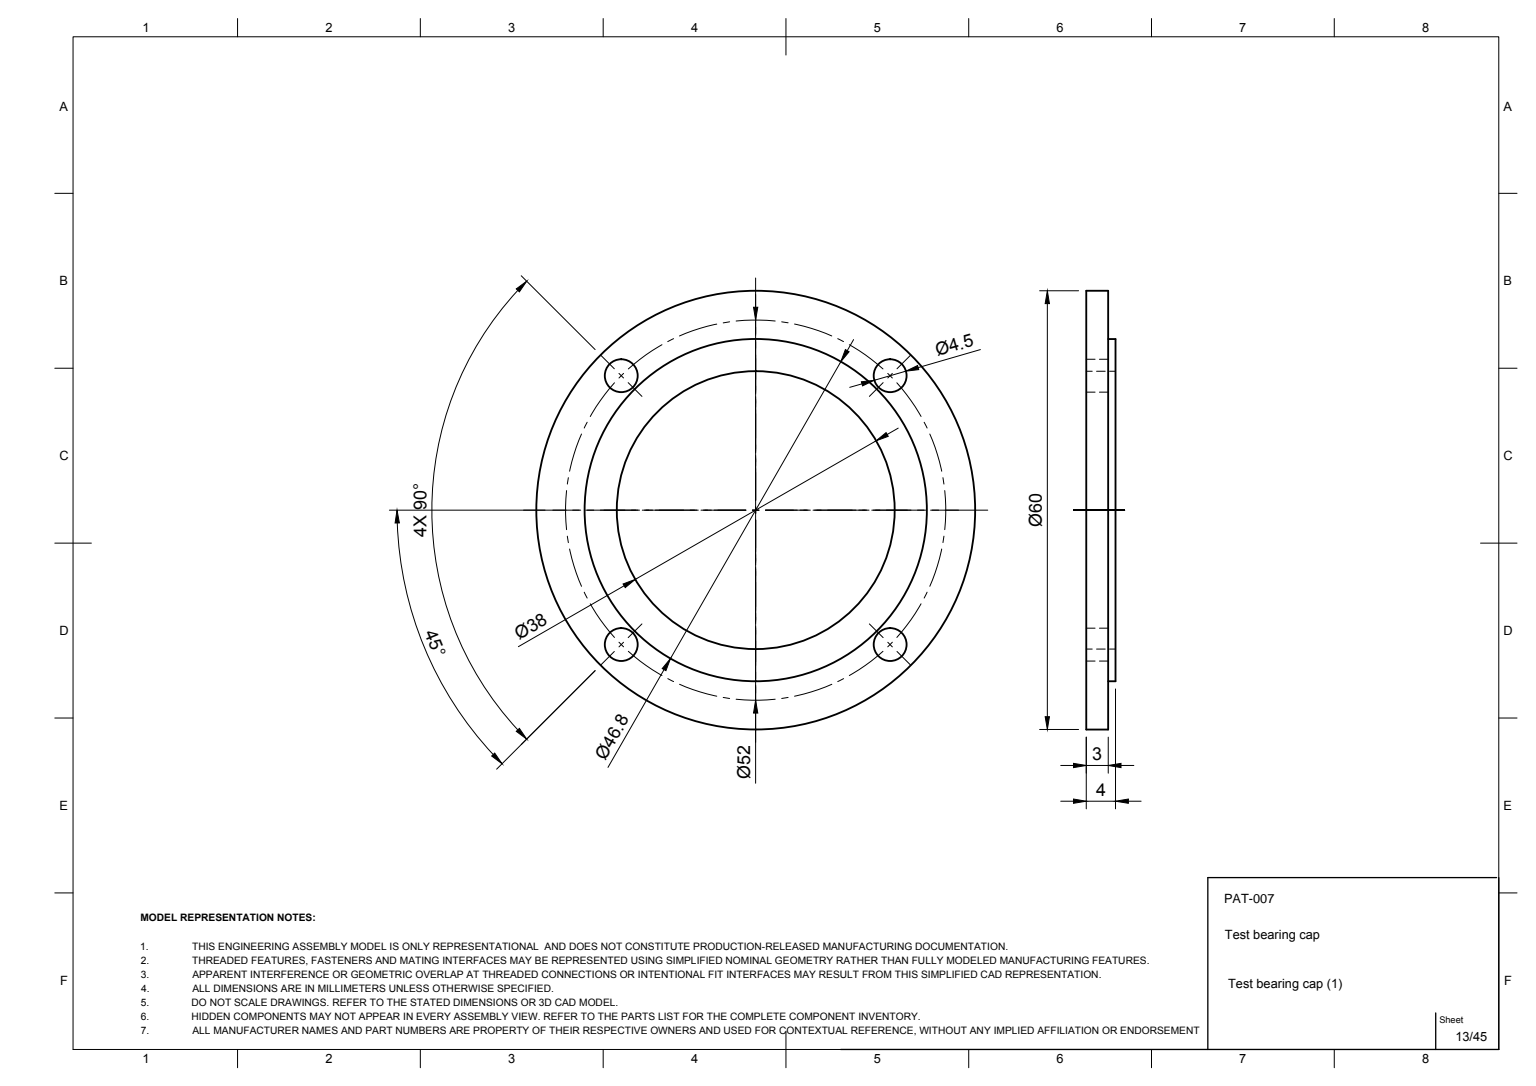
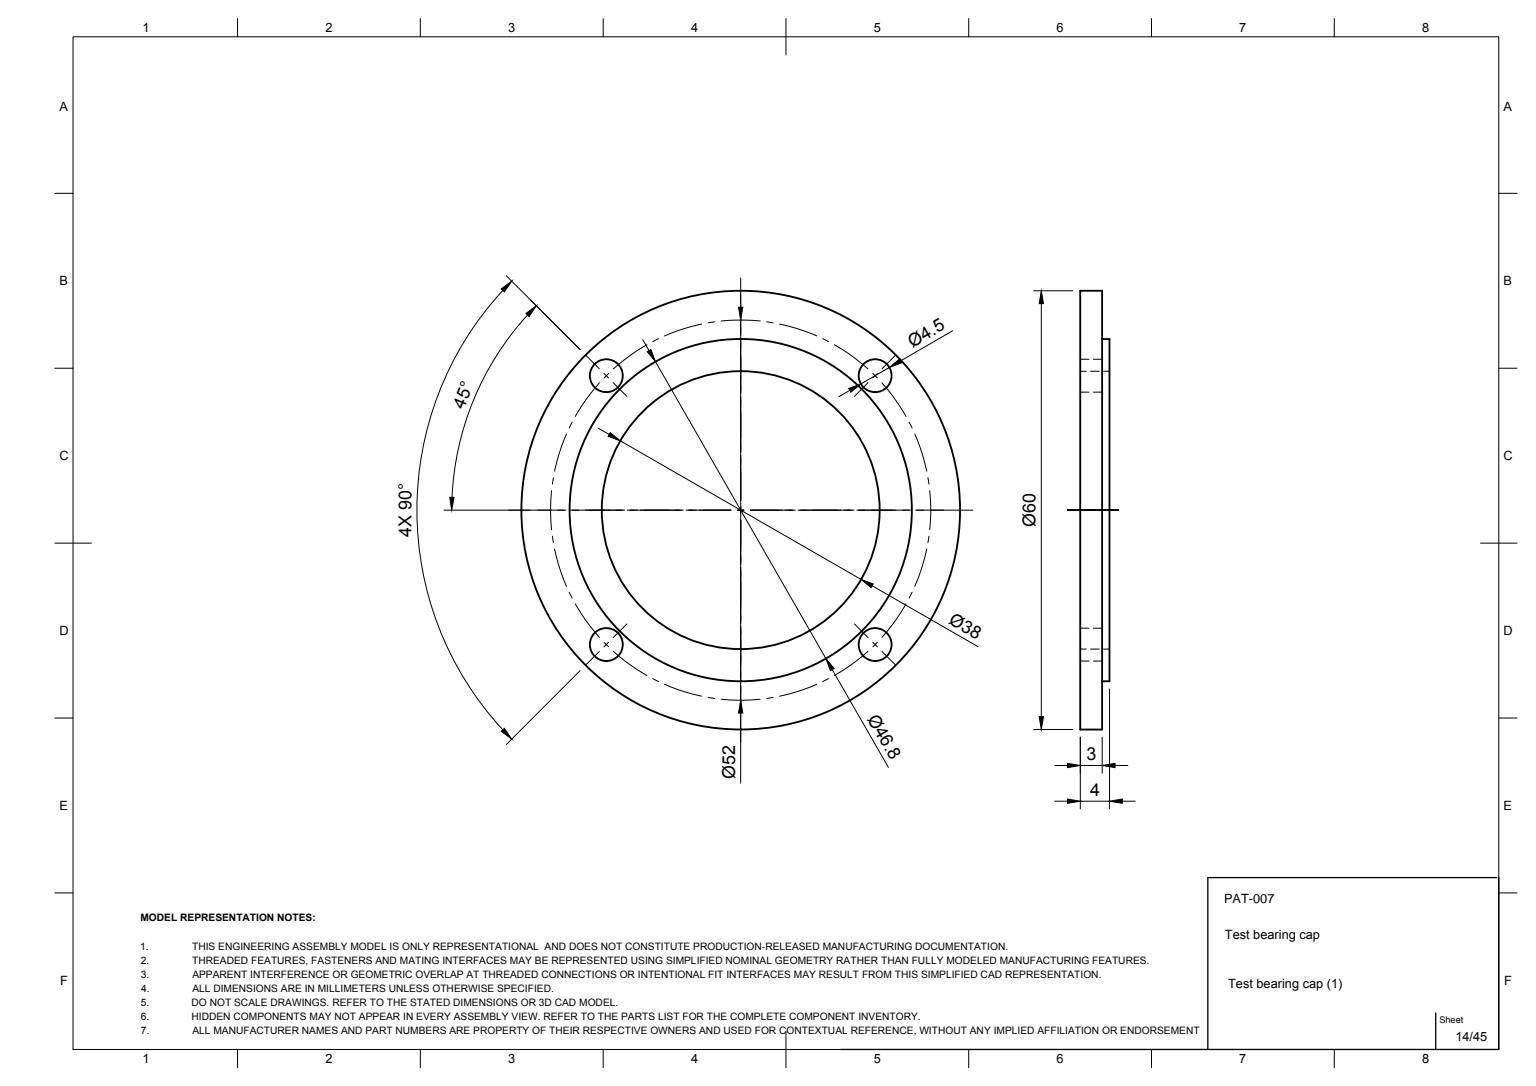
ISO-10303-21;
HEADER;
/* Generated by software containing ST-Developer
 * from STEP Tools, Inc. (www.steptools.com) 
 */

FILE_DESCRIPTION(
/* description */ ('Bearing friction torque test rig'),
/* implementation_level */ '2;1');

FILE_NAME(
/* name */ 'Test bearing cap.step',
/* time_stamp */ '2026-10-28T03:24:04-07:00',
/* author */ (''),
/* organization */ (''),
/* preprocessor_version */ 'ST-DEVELOPER v20.2',
/* originating_system */ 'Autodesk Translation Framework v15.17.0.0',
/* authorisation */ '');

FILE_SCHEMA (('AUTOMOTIVE_DESIGN { 1 0 10303 214 3 1 1 }'));
ENDSEC;

DATA;
#10=MECHANICAL_DESIGN_GEOMETRIC_PRESENTATION_REPRESENTATION('',(#547),#14822);
#469=SHAPE_REPRESENTATION_RELATIONSHIP('SRR','None',#15008,#508);
#508=ADVANCED_BREP_SHAPE_REPRESENTATION('',(#601),#14788);
#547=STYLED_ITEM('',(#15284),#601);
#601=MANIFOLD_SOLID_BREP('Body1',#7663);
#755=FACE_BOUND('',#1774,.T.);
#756=FACE_BOUND('',#1778,.T.);
#757=FACE_BOUND('',#1779,.T.);
#758=FACE_BOUND('',#1780,.T.);
#759=FACE_BOUND('',#1781,.T.);
#760=FACE_BOUND('',#1782,.T.);
#761=FACE_BOUND('',#1784,.T.);
#762=FACE_BOUND('',#1785,.T.);
#763=FACE_BOUND('',#1786,.T.);
#764=FACE_BOUND('',#1787,.T.);
#765=FACE_BOUND('',#1788,.T.);
#921=PLANE('',#8423);
#922=PLANE('',#8430);
#923=PLANE('',#8431);
#1212=FACE_OUTER_BOUND('',#1768,.T.);
#1213=FACE_OUTER_BOUND('',#1769,.T.);
#1214=FACE_OUTER_BOUND('',#1770,.T.);
#1215=FACE_OUTER_BOUND('',#1771,.T.);
#1216=FACE_OUTER_BOUND('',#1772,.T.);
#1217=FACE_OUTER_BOUND('',#1773,.T.);
#1218=FACE_OUTER_BOUND('',#1775,.T.);
#1219=FACE_OUTER_BOUND('',#1776,.T.);
#1220=FACE_OUTER_BOUND('',#1777,.T.);
#1221=FACE_OUTER_BOUND('',#1783,.T.);
#1768=EDGE_LOOP('',(#5676,#5677,#5678,#5679));
#1769=EDGE_LOOP('',(#5680,#5681,#5682,#5683));
#1770=EDGE_LOOP('',(#5684,#5685,#5686,#5687));
#1771=EDGE_LOOP('',(#5688,#5689,#5690,#5691));
#1772=EDGE_LOOP('',(#5692,#5693,#5694,#5695));
#1773=EDGE_LOOP('',(#5696));
#1774=EDGE_LOOP('',(#5697));
#1775=EDGE_LOOP('',(#5698,#5699,#5700,#5701));
#1776=EDGE_LOOP('',(#5702,#5703,#5704,#5705));
#1777=EDGE_LOOP('',(#5706));
#1778=EDGE_LOOP('',(#5707));
#1779=EDGE_LOOP('',(#5708));
#1780=EDGE_LOOP('',(#5709));
#1781=EDGE_LOOP('',(#5710));
#1782=EDGE_LOOP('',(#5711));
#1783=EDGE_LOOP('',(#5712));
#1784=EDGE_LOOP('',(#5713));
#1785=EDGE_LOOP('',(#5714));
#1786=EDGE_LOOP('',(#5715));
#1787=EDGE_LOOP('',(#5716));
#1788=EDGE_LOOP('',(#5717));
#2341=LINE('',#12226,#2785);
#2342=LINE('',#12232,#2786);
#2343=LINE('',#12238,#2787);
#2344=LINE('',#12244,#2788);
#2345=LINE('',#12250,#2789);
#2346=LINE('',#12257,#2790);
#2347=LINE('',#12263,#2791);
#2785=VECTOR('',#9824,0.225);
#2786=VECTOR('',#9831,0.225);
#2787=VECTOR('',#9838,0.225);
#2788=VECTOR('',#9845,0.225);
#2789=VECTOR('',#9852,2.34);
#2790=VECTOR('',#9861,1.9);
#2791=VECTOR('',#9868,3.);
#3243=CIRCLE('',#8409,0.225);
#3244=CIRCLE('',#8410,0.225);
#3245=CIRCLE('',#8412,0.225);
#3246=CIRCLE('',#8413,0.225);
#3247=CIRCLE('',#8415,0.225);
#3248=CIRCLE('',#8416,0.225);
#3249=CIRCLE('',#8418,0.225);
#3250=CIRCLE('',#8419,0.225);
#3251=CIRCLE('',#8421,2.34);
#3252=CIRCLE('',#8422,2.34);
#3253=CIRCLE('',#8424,1.9);
#3254=CIRCLE('',#8426,1.9);
#3255=CIRCLE('',#8428,3.);
#3256=CIRCLE('',#8429,3.);
#3729=VERTEX_POINT('',#12223);
#3730=VERTEX_POINT('',#12225);
#3731=VERTEX_POINT('',#12229);
#3732=VERTEX_POINT('',#12231);
#3733=VERTEX_POINT('',#12235);
#3734=VERTEX_POINT('',#12237);
#3735=VERTEX_POINT('',#12241);
#3736=VERTEX_POINT('',#12243);
#3737=VERTEX_POINT('',#12247);
#3738=VERTEX_POINT('',#12249);
#3739=VERTEX_POINT('',#12253);
#3740=VERTEX_POINT('',#12256);
#3741=VERTEX_POINT('',#12260);
#3742=VERTEX_POINT('',#12262);
#4464=EDGE_CURVE('',#3729,#3729,#3243,.T.);
#4465=EDGE_CURVE('',#3729,#3730,#2341,.T.);
#4466=EDGE_CURVE('',#3730,#3730,#3244,.T.);
#4467=EDGE_CURVE('',#3731,#3731,#3245,.T.);
#4468=EDGE_CURVE('',#3731,#3732,#2342,.T.);
#4469=EDGE_CURVE('',#3732,#3732,#3246,.T.);
#4470=EDGE_CURVE('',#3733,#3733,#3247,.T.);
#4471=EDGE_CURVE('',#3733,#3734,#2343,.T.);
#4472=EDGE_CURVE('',#3734,#3734,#3248,.T.);
#4473=EDGE_CURVE('',#3735,#3735,#3249,.T.);
#4474=EDGE_CURVE('',#3735,#3736,#2344,.T.);
#4475=EDGE_CURVE('',#3736,#3736,#3250,.T.);
#4476=EDGE_CURVE('',#3737,#3737,#3251,.T.);
#4477=EDGE_CURVE('',#3737,#3738,#2345,.T.);
#4478=EDGE_CURVE('',#3738,#3738,#3252,.T.);
#4479=EDGE_CURVE('',#3739,#3739,#3253,.T.);
#4480=EDGE_CURVE('',#3739,#3740,#2346,.T.);
#4481=EDGE_CURVE('',#3740,#3740,#3254,.T.);
#4482=EDGE_CURVE('',#3741,#3741,#3255,.T.);
#4483=EDGE_CURVE('',#3741,#3742,#2347,.T.);
#4484=EDGE_CURVE('',#3742,#3742,#3256,.T.);
#5676=ORIENTED_EDGE('',*,*,#4464,.F.);
#5677=ORIENTED_EDGE('',*,*,#4465,.T.);
#5678=ORIENTED_EDGE('',*,*,#4466,.F.);
#5679=ORIENTED_EDGE('',*,*,#4465,.F.);
#5680=ORIENTED_EDGE('',*,*,#4467,.F.);
#5681=ORIENTED_EDGE('',*,*,#4468,.T.);
#5682=ORIENTED_EDGE('',*,*,#4469,.F.);
#5683=ORIENTED_EDGE('',*,*,#4468,.F.);
#5684=ORIENTED_EDGE('',*,*,#4470,.F.);
#5685=ORIENTED_EDGE('',*,*,#4471,.T.);
#5686=ORIENTED_EDGE('',*,*,#4472,.F.);
#5687=ORIENTED_EDGE('',*,*,#4471,.F.);
#5688=ORIENTED_EDGE('',*,*,#4473,.F.);
#5689=ORIENTED_EDGE('',*,*,#4474,.T.);
#5690=ORIENTED_EDGE('',*,*,#4475,.F.);
#5691=ORIENTED_EDGE('',*,*,#4474,.F.);
#5692=ORIENTED_EDGE('',*,*,#4476,.F.);
#5693=ORIENTED_EDGE('',*,*,#4477,.T.);
#5694=ORIENTED_EDGE('',*,*,#4478,.F.);
#5695=ORIENTED_EDGE('',*,*,#4477,.F.);
#5696=ORIENTED_EDGE('',*,*,#4476,.T.);
#5697=ORIENTED_EDGE('',*,*,#4479,.T.);
#5698=ORIENTED_EDGE('',*,*,#4479,.F.);
#5699=ORIENTED_EDGE('',*,*,#4480,.T.);
#5700=ORIENTED_EDGE('',*,*,#4481,.T.);
#5701=ORIENTED_EDGE('',*,*,#4480,.F.);
#5702=ORIENTED_EDGE('',*,*,#4482,.F.);
#5703=ORIENTED_EDGE('',*,*,#4483,.T.);
#5704=ORIENTED_EDGE('',*,*,#4484,.T.);
#5705=ORIENTED_EDGE('',*,*,#4483,.F.);
#5706=ORIENTED_EDGE('',*,*,#4482,.T.);
#5707=ORIENTED_EDGE('',*,*,#4478,.T.);
#5708=ORIENTED_EDGE('',*,*,#4475,.T.);
#5709=ORIENTED_EDGE('',*,*,#4472,.T.);
#5710=ORIENTED_EDGE('',*,*,#4469,.T.);
#5711=ORIENTED_EDGE('',*,*,#4466,.T.);
#5712=ORIENTED_EDGE('',*,*,#4484,.F.);
#5713=ORIENTED_EDGE('',*,*,#4481,.F.);
#5714=ORIENTED_EDGE('',*,*,#4473,.T.);
#5715=ORIENTED_EDGE('',*,*,#4470,.T.);
#5716=ORIENTED_EDGE('',*,*,#4467,.T.);
#5717=ORIENTED_EDGE('',*,*,#4464,.T.);
#7110=CYLINDRICAL_SURFACE('',#8408,0.225);
#7111=CYLINDRICAL_SURFACE('',#8411,0.225);
#7112=CYLINDRICAL_SURFACE('',#8414,0.225);
#7113=CYLINDRICAL_SURFACE('',#8417,0.225);
#7114=CYLINDRICAL_SURFACE('',#8420,2.34);
#7115=CYLINDRICAL_SURFACE('',#8425,1.9);
#7116=CYLINDRICAL_SURFACE('',#8427,3.);
#7323=ADVANCED_FACE('',(#1212),#7110,.F.);
#7324=ADVANCED_FACE('',(#1213),#7111,.F.);
#7325=ADVANCED_FACE('',(#1214),#7112,.F.);
#7326=ADVANCED_FACE('',(#1215),#7113,.F.);
#7327=ADVANCED_FACE('',(#1216),#7114,.T.);
#7328=ADVANCED_FACE('',(#1217,#755),#921,.T.);
#7329=ADVANCED_FACE('',(#1218),#7115,.F.);
#7330=ADVANCED_FACE('',(#1219),#7116,.T.);
#7331=ADVANCED_FACE('',(#1220,#756,#757,#758,#759,#760),#922,.T.);
#7332=ADVANCED_FACE('',(#1221,#761,#762,#763,#764,#765),#923,.F.);
#7663=CLOSED_SHELL('',(#7323,#7324,#7325,#7326,#7327,#7328,#7329,#7330,
#7331,#7332));
#8407=AXIS2_PLACEMENT_3D('',#12221,#9818,#9819);
#8408=AXIS2_PLACEMENT_3D('',#12222,#9820,#9821);
#8409=AXIS2_PLACEMENT_3D('',#12224,#9822,#9823);
#8410=AXIS2_PLACEMENT_3D('',#12227,#9825,#9826);
#8411=AXIS2_PLACEMENT_3D('',#12228,#9827,#9828);
#8412=AXIS2_PLACEMENT_3D('',#12230,#9829,#9830);
#8413=AXIS2_PLACEMENT_3D('',#12233,#9832,#9833);
#8414=AXIS2_PLACEMENT_3D('',#12234,#9834,#9835);
#8415=AXIS2_PLACEMENT_3D('',#12236,#9836,#9837);
#8416=AXIS2_PLACEMENT_3D('',#12239,#9839,#9840);
#8417=AXIS2_PLACEMENT_3D('',#12240,#9841,#9842);
#8418=AXIS2_PLACEMENT_3D('',#12242,#9843,#9844);
#8419=AXIS2_PLACEMENT_3D('',#12245,#9846,#9847);
#8420=AXIS2_PLACEMENT_3D('',#12246,#9848,#9849);
#8421=AXIS2_PLACEMENT_3D('',#12248,#9850,#9851);
#8422=AXIS2_PLACEMENT_3D('',#12251,#9853,#9854);
#8423=AXIS2_PLACEMENT_3D('',#12252,#9855,#9856);
#8424=AXIS2_PLACEMENT_3D('',#12254,#9857,#9858);
#8425=AXIS2_PLACEMENT_3D('',#12255,#9859,#9860);
#8426=AXIS2_PLACEMENT_3D('',#12258,#9862,#9863);
#8427=AXIS2_PLACEMENT_3D('',#12259,#9864,#9865);
#8428=AXIS2_PLACEMENT_3D('',#12261,#9866,#9867);
#8429=AXIS2_PLACEMENT_3D('',#12264,#9869,#9870);
#8430=AXIS2_PLACEMENT_3D('',#12265,#9871,#9872);
#8431=AXIS2_PLACEMENT_3D('',#12266,#9873,#9874);
#9818=DIRECTION('axis',(0.,0.,1.));
#9819=DIRECTION('refdir',(1.,0.,0.));
#9820=DIRECTION('center_axis',(0.,1.,0.));
#9821=DIRECTION('ref_axis',(1.,0.,0.));
#9822=DIRECTION('center_axis',(0.,1.,0.));
#9823=DIRECTION('ref_axis',(1.,0.,0.));
#9824=DIRECTION('',(0.,1.,0.));
#9825=DIRECTION('center_axis',(0.,-1.,0.));
#9826=DIRECTION('ref_axis',(1.,0.,0.));
#9827=DIRECTION('center_axis',(0.,1.,0.));
#9828=DIRECTION('ref_axis',(1.,0.,0.));
#9829=DIRECTION('center_axis',(0.,1.,0.));
#9830=DIRECTION('ref_axis',(1.,0.,0.));
#9831=DIRECTION('',(0.,1.,0.));
#9832=DIRECTION('center_axis',(0.,-1.,0.));
#9833=DIRECTION('ref_axis',(1.,0.,0.));
#9834=DIRECTION('center_axis',(0.,1.,0.));
#9835=DIRECTION('ref_axis',(1.,0.,0.));
#9836=DIRECTION('center_axis',(0.,1.,0.));
#9837=DIRECTION('ref_axis',(1.,0.,0.));
#9838=DIRECTION('',(0.,1.,0.));
#9839=DIRECTION('center_axis',(0.,-1.,0.));
#9840=DIRECTION('ref_axis',(1.,0.,0.));
#9841=DIRECTION('center_axis',(0.,1.,0.));
#9842=DIRECTION('ref_axis',(1.,0.,0.));
#9843=DIRECTION('center_axis',(0.,1.,0.));
#9844=DIRECTION('ref_axis',(1.,0.,0.));
#9845=DIRECTION('',(0.,1.,0.));
#9846=DIRECTION('center_axis',(0.,-1.,0.));
#9847=DIRECTION('ref_axis',(1.,0.,0.));
#9848=DIRECTION('center_axis',(0.,1.,0.));
#9849=DIRECTION('ref_axis',(1.,0.,0.));
#9850=DIRECTION('center_axis',(0.,1.,0.));
#9851=DIRECTION('ref_axis',(1.,0.,0.));
#9852=DIRECTION('',(0.,-1.,0.));
#9853=DIRECTION('center_axis',(0.,-1.,0.));
#9854=DIRECTION('ref_axis',(1.,0.,0.));
#9855=DIRECTION('center_axis',(0.,1.,0.));
#9856=DIRECTION('ref_axis',(1.,0.,0.));
#9857=DIRECTION('center_axis',(0.,-1.,0.));
#9858=DIRECTION('ref_axis',(1.,0.,0.));
#9859=DIRECTION('center_axis',(0.,1.,0.));
#9860=DIRECTION('ref_axis',(1.,0.,0.));
#9861=DIRECTION('',(0.,-1.,0.));
#9862=DIRECTION('center_axis',(0.,-1.,0.));
#9863=DIRECTION('ref_axis',(1.,0.,0.));
#9864=DIRECTION('center_axis',(0.,1.,0.));
#9865=DIRECTION('ref_axis',(1.,0.,0.));
#9866=DIRECTION('center_axis',(0.,1.,0.));
#9867=DIRECTION('ref_axis',(1.,0.,0.));
#9868=DIRECTION('',(0.,-1.,0.));
#9869=DIRECTION('center_axis',(0.,1.,0.));
#9870=DIRECTION('ref_axis',(1.,0.,0.));
#9871=DIRECTION('center_axis',(0.,1.,0.));
#9872=DIRECTION('ref_axis',(1.,0.,0.));
#9873=DIRECTION('center_axis',(0.,1.,0.));
#9874=DIRECTION('ref_axis',(1.,0.,0.));
#12221=CARTESIAN_POINT('',(0.,0.,0.));
#12222=CARTESIAN_POINT('Origin',(-1.83847763108502,-1.2,5.16152236891498));
#12223=CARTESIAN_POINT('',(-2.06347763108502,-1.1,5.16152236891498));
#12224=CARTESIAN_POINT('Origin',(-1.83847763108502,-1.1,5.16152236891498));
#12225=CARTESIAN_POINT('',(-2.06347763108502,-0.8,5.16152236891498));
#12226=CARTESIAN_POINT('',(-2.06347763108502,-1.2,5.16152236891498));
#12227=CARTESIAN_POINT('Origin',(-1.83847763108502,-0.8,5.16152236891498));
#12228=CARTESIAN_POINT('Origin',(-1.83847763108502,-1.2,8.83847763108502));
#12229=CARTESIAN_POINT('',(-2.06347763108502,-1.1,8.83847763108502));
#12230=CARTESIAN_POINT('Origin',(-1.83847763108502,-1.1,8.83847763108502));
#12231=CARTESIAN_POINT('',(-2.06347763108502,-0.8,8.83847763108502));
#12232=CARTESIAN_POINT('',(-2.06347763108502,-1.2,8.83847763108502));
#12233=CARTESIAN_POINT('Origin',(-1.83847763108502,-0.8,8.83847763108502));
#12234=CARTESIAN_POINT('Origin',(1.83847763108502,-1.2,8.83847763108502));
#12235=CARTESIAN_POINT('',(1.61347763108502,-1.1,8.83847763108502));
#12236=CARTESIAN_POINT('Origin',(1.83847763108502,-1.1,8.83847763108502));
#12237=CARTESIAN_POINT('',(1.61347763108502,-0.8,8.83847763108502));
#12238=CARTESIAN_POINT('',(1.61347763108502,-1.2,8.83847763108502));
#12239=CARTESIAN_POINT('Origin',(1.83847763108502,-0.8,8.83847763108502));
#12240=CARTESIAN_POINT('Origin',(1.83847763108502,-1.2,5.16152236891498));
#12241=CARTESIAN_POINT('',(1.61347763108502,-1.1,5.16152236891498));
#12242=CARTESIAN_POINT('Origin',(1.83847763108502,-1.1,5.16152236891498));
#12243=CARTESIAN_POINT('',(1.61347763108502,-0.8,5.16152236891498));
#12244=CARTESIAN_POINT('',(1.61347763108502,-1.2,5.16152236891498));
#12245=CARTESIAN_POINT('Origin',(1.83847763108502,-0.8,5.16152236891498));
#12246=CARTESIAN_POINT('Origin',(0.,-0.8,7.));
#12247=CARTESIAN_POINT('',(-2.34,-0.7,7.));
#12248=CARTESIAN_POINT('Origin',(0.,-0.7,7.));
#12249=CARTESIAN_POINT('',(-2.34,-0.8,7.));
#12250=CARTESIAN_POINT('',(-2.34,-0.8,7.));
#12251=CARTESIAN_POINT('Origin',(0.,-0.8,7.));
#12252=CARTESIAN_POINT('Origin',(0.,-0.7,7.));
#12253=CARTESIAN_POINT('',(-1.9,-0.7,7.));
#12254=CARTESIAN_POINT('Origin',(0.,-0.7,7.));
#12255=CARTESIAN_POINT('Origin',(0.,-1.1,7.));
#12256=CARTESIAN_POINT('',(-1.9,-1.1,7.));
#12257=CARTESIAN_POINT('',(-1.9,-1.1,7.));
#12258=CARTESIAN_POINT('Origin',(0.,-1.1,7.));
#12259=CARTESIAN_POINT('Origin',(0.,-1.1,7.));
#12260=CARTESIAN_POINT('',(-3.,-0.8,7.));
#12261=CARTESIAN_POINT('Origin',(0.,-0.8,7.));
#12262=CARTESIAN_POINT('',(-3.,-1.1,7.));
#12263=CARTESIAN_POINT('',(-3.,-1.1,7.));
#12264=CARTESIAN_POINT('Origin',(0.,-1.1,7.));
#12265=CARTESIAN_POINT('Origin',(0.,-0.8,7.));
#12266=CARTESIAN_POINT('Origin',(0.,-1.1,7.));
#14743=UNCERTAINTY_MEASURE_WITH_UNIT(LENGTH_MEASURE(0.001),#14823,
'DISTANCE_ACCURACY_VALUE',
'Maximum model space distance between geometric entities at asserted c
onnectivities');
#14777=UNCERTAINTY_MEASURE_WITH_UNIT(LENGTH_MEASURE(0.001),#14823,
'DISTANCE_ACCURACY_VALUE',
'Maximum model space distance between geometric entities at asserted c
onnectivities');
#14788=(
GEOMETRIC_REPRESENTATION_CONTEXT(3)
GLOBAL_UNCERTAINTY_ASSIGNED_CONTEXT((#14743))
GLOBAL_UNIT_ASSIGNED_CONTEXT((#14823,#14825,#14826))
REPRESENTATION_CONTEXT('','3D')
);
#14822=(
GEOMETRIC_REPRESENTATION_CONTEXT(3)
GLOBAL_UNCERTAINTY_ASSIGNED_CONTEXT((#14777))
GLOBAL_UNIT_ASSIGNED_CONTEXT((#14823,#14825,#14826))
REPRESENTATION_CONTEXT('','3D')
);
#14823=(
LENGTH_UNIT()
NAMED_UNIT(*)
SI_UNIT(.CENTI.,.METRE.)
);
#14825=(
NAMED_UNIT(*)
PLANE_ANGLE_UNIT()
SI_UNIT($,.RADIAN.)
);
#14826=(
NAMED_UNIT(*)
SI_UNIT($,.STERADIAN.)
SOLID_ANGLE_UNIT()
);
#14837=SHAPE_DEFINITION_REPRESENTATION(#14881,#15008);
#14881=PRODUCT_DEFINITION_SHAPE('',$,#15053);
#15008=SHAPE_REPRESENTATION('',(#8407),#14788);
#15042=PRODUCT_DEFINITION_CONTEXT('part definition',#15176,'design');
#15053=PRODUCT_DEFINITION('Test bearing cap','Test bearing cap',#15097,
#15042);
#15097=PRODUCT_DEFINITION_FORMATION('',$,#15188);
#15176=APPLICATION_CONTEXT(
'Core Data for Automotive Mechanical Design Process');
#15177=PRODUCT_CONTEXT('part definition',#15176,'mechanical');
#15188=PRODUCT('Test bearing cap','Test bearing cap','Test bearing cap',
(#15177));
#15278=COLOUR_RGB('Grey',0.48,0.52,0.57);
#15279=FILL_AREA_STYLE_COLOUR('',#15278);
#15280=FILL_AREA_STYLE('',(#15279));
#15281=SURFACE_STYLE_FILL_AREA(#15280);
#15282=SURFACE_SIDE_STYLE('',(#15281));
#15283=SURFACE_STYLE_USAGE(.BOTH.,#15282);
#15284=PRESENTATION_STYLE_ASSIGNMENT((#15283));
ENDSEC;
END-ISO-10303-21;
